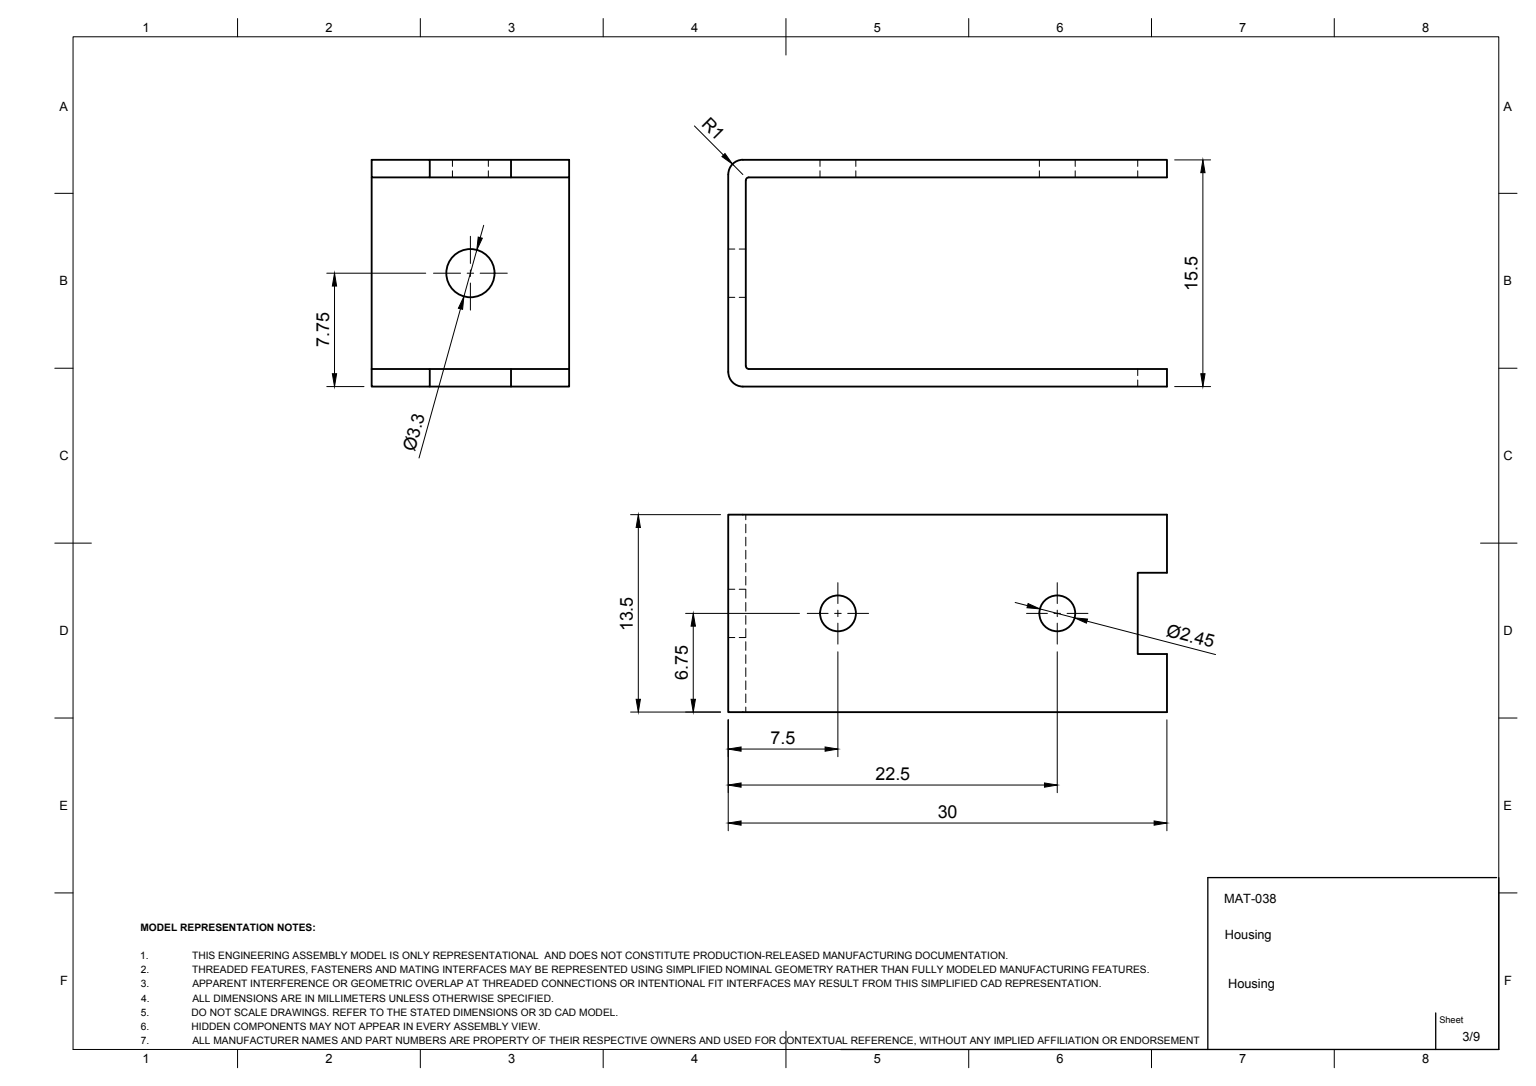
ISO-10303-21;
HEADER;
/* Generated by software containing ST-Developer
 * from STEP Tools, Inc. (www.steptools.com) 
 */

FILE_DESCRIPTION(
/* description */ ('STEP AP214'),
/* implementation_level */ '2;1');

FILE_NAME(
/* name */ 'Housing.step',
/* time_stamp */ '2026-11-14T21:32:33-08:00',
/* author */ (''),
/* organization */ (''),
/* preprocessor_version */ 'ST-DEVELOPER v20.2',
/* originating_system */ 'Autodesk Translation Framework v15.17.0.0',
/* authorisation */ '');

FILE_SCHEMA (('AUTOMOTIVE_DESIGN { 1 0 10303 214 3 1 1 }'));
ENDSEC;

DATA;
#10=MECHANICAL_DESIGN_GEOMETRIC_PRESENTATION_REPRESENTATION('',(#177),#10551);
#159=SHAPE_REPRESENTATION_RELATIONSHIP('SRR','None',#10586,#168);
#168=ADVANCED_BREP_SHAPE_REPRESENTATION('',(#187),#10542);
#177=STYLED_ITEM('',(#10640),#187);
#187=MANIFOLD_SOLID_BREP('Body1',#3426);
#197=FACE_BOUND('',#522,.T.);
#198=FACE_BOUND('',#523,.T.);
#199=FACE_BOUND('',#525,.T.);
#200=FACE_BOUND('',#531,.T.);
#201=FACE_BOUND('',#533,.T.);
#202=FACE_BOUND('',#534,.T.);
#224=PLANE('',#3547);
#225=PLANE('',#3548);
#226=PLANE('',#3549);
#227=PLANE('',#3550);
#228=PLANE('',#3551);
#229=PLANE('',#3552);
#230=PLANE('',#3553);
#231=PLANE('',#3554);
#232=PLANE('',#3559);
#233=PLANE('',#3564);
#234=PLANE('',#3565);
#235=PLANE('',#3566);
#236=PLANE('',#3571);
#237=PLANE('',#3572);
#238=PLANE('',#3573);
#239=PLANE('',#3574);
#240=PLANE('',#3575);
#241=PLANE('',#3576);
#294=FACE_OUTER_BOUND('',#514,.T.);
#295=FACE_OUTER_BOUND('',#515,.T.);
#296=FACE_OUTER_BOUND('',#516,.T.);
#297=FACE_OUTER_BOUND('',#517,.T.);
#298=FACE_OUTER_BOUND('',#518,.T.);
#299=FACE_OUTER_BOUND('',#519,.T.);
#300=FACE_OUTER_BOUND('',#520,.T.);
#301=FACE_OUTER_BOUND('',#521,.T.);
#302=FACE_OUTER_BOUND('',#524,.T.);
#303=FACE_OUTER_BOUND('',#526,.T.);
#304=FACE_OUTER_BOUND('',#527,.T.);
#305=FACE_OUTER_BOUND('',#528,.T.);
#306=FACE_OUTER_BOUND('',#529,.T.);
#307=FACE_OUTER_BOUND('',#530,.T.);
#308=FACE_OUTER_BOUND('',#532,.T.);
#309=FACE_OUTER_BOUND('',#535,.T.);
#310=FACE_OUTER_BOUND('',#536,.T.);
#311=FACE_OUTER_BOUND('',#537,.T.);
#312=FACE_OUTER_BOUND('',#538,.T.);
#313=FACE_OUTER_BOUND('',#539,.T.);
#314=FACE_OUTER_BOUND('',#540,.T.);
#315=FACE_OUTER_BOUND('',#541,.T.);
#316=FACE_OUTER_BOUND('',#542,.T.);
#317=FACE_OUTER_BOUND('',#543,.T.);
#318=FACE_OUTER_BOUND('',#544,.T.);
#514=EDGE_LOOP('',(#2188,#2189,#2190,#2191));
#515=EDGE_LOOP('',(#2192,#2193,#2194,#2195));
#516=EDGE_LOOP('',(#2196,#2197,#2198,#2199));
#517=EDGE_LOOP('',(#2200,#2201,#2202,#2203));
#518=EDGE_LOOP('',(#2204,#2205,#2206,#2207));
#519=EDGE_LOOP('',(#2208,#2209,#2210,#2211));
#520=EDGE_LOOP('',(#2212,#2213,#2214,#2215));
#521=EDGE_LOOP('',(#2216,#2217,#2218,#2219,#2220,#2221,#2222,#2223));
#522=EDGE_LOOP('',(#2224));
#523=EDGE_LOOP('',(#2225));
#524=EDGE_LOOP('',(#2226,#2227,#2228,#2229));
#525=EDGE_LOOP('',(#2230));
#526=EDGE_LOOP('',(#2231,#2232,#2233,#2234,#2235,#2236,#2237,#2238));
#527=EDGE_LOOP('',(#2239,#2240,#2241,#2242,#2243,#2244,#2245,#2246,#2247,
#2248,#2249,#2250));
#528=EDGE_LOOP('',(#2251,#2252,#2253,#2254,#2255,#2256,#2257,#2258,#2259,
#2260,#2261,#2262));
#529=EDGE_LOOP('',(#2263,#2264,#2265,#2266,#2267,#2268,#2269,#2270));
#530=EDGE_LOOP('',(#2271,#2272,#2273,#2274));
#531=EDGE_LOOP('',(#2275));
#532=EDGE_LOOP('',(#2276,#2277,#2278,#2279,#2280,#2281,#2282,#2283));
#533=EDGE_LOOP('',(#2284));
#534=EDGE_LOOP('',(#2285));
#535=EDGE_LOOP('',(#2286,#2287,#2288,#2289));
#536=EDGE_LOOP('',(#2290,#2291,#2292,#2293));
#537=EDGE_LOOP('',(#2294,#2295,#2296,#2297));
#538=EDGE_LOOP('',(#2298,#2299,#2300,#2301));
#539=EDGE_LOOP('',(#2302,#2303,#2304,#2305));
#540=EDGE_LOOP('',(#2306,#2307,#2308,#2309));
#541=EDGE_LOOP('',(#2310,#2311,#2312,#2313));
#542=EDGE_LOOP('',(#2314,#2315,#2316,#2317));
#543=EDGE_LOOP('',(#2318,#2319,#2320,#2321));
#544=EDGE_LOOP('',(#2322,#2323,#2324,#2325));
#761=LINE('',#5239,#958);
#762=LINE('',#5245,#959);
#763=LINE('',#5251,#960);
#764=LINE('',#5256,#961);
#765=LINE('',#5258,#962);
#766=LINE('',#5260,#963);
#767=LINE('',#5261,#964);
#768=LINE('',#5265,#965);
#769=LINE('',#5267,#966);
#770=LINE('',#5269,#967);
#771=LINE('',#5270,#968);
#772=LINE('',#5274,#969);
#773=LINE('',#5276,#970);
#774=LINE('',#5278,#971);
#775=LINE('',#5279,#972);
#776=LINE('',#5283,#973);
#777=LINE('',#5285,#974);
#778=LINE('',#5287,#975);
#779=LINE('',#5288,#976);
#780=LINE('',#5291,#977);
#781=LINE('',#5293,#978);
#782=LINE('',#5294,#979);
#783=LINE('',#5296,#980);
#784=LINE('',#5298,#981);
#785=LINE('',#5299,#982);
#786=LINE('',#5303,#983);
#787=LINE('',#5305,#984);
#788=LINE('',#5307,#985);
#789=LINE('',#5308,#986);
#790=LINE('',#5312,#987);
#791=LINE('',#5313,#988);
#792=LINE('',#5315,#989);
#793=LINE('',#5317,#990);
#794=LINE('',#5318,#991);
#795=LINE('',#5319,#992);
#796=LINE('',#5324,#993);
#797=LINE('',#5328,#994);
#798=LINE('',#5331,#995);
#799=LINE('',#5335,#996);
#800=LINE('',#5339,#997);
#801=LINE('',#5342,#998);
#802=LINE('',#5346,#999);
#803=LINE('',#5348,#1000);
#804=LINE('',#5349,#1001);
#805=LINE('',#5350,#1002);
#806=LINE('',#5352,#1003);
#807=LINE('',#5353,#1004);
#808=LINE('',#5357,#1005);
#809=LINE('',#5358,#1006);
#810=LINE('',#5359,#1007);
#811=LINE('',#5360,#1008);
#812=LINE('',#5366,#1009);
#813=LINE('',#5368,#1010);
#814=LINE('',#5371,#1011);
#815=LINE('',#5373,#1012);
#958=VECTOR('',#4044,1.225);
#959=VECTOR('',#4051,1.225);
#960=VECTOR('',#4058,1.65);
#961=VECTOR('',#4063,1000.);
#962=VECTOR('',#4064,1000.);
#963=VECTOR('',#4065,1000.);
#964=VECTOR('',#4066,1000.);
#965=VECTOR('',#4069,1000.);
#966=VECTOR('',#4070,1000.);
#967=VECTOR('',#4071,1000.);
#968=VECTOR('',#4072,1000.);
#969=VECTOR('',#4075,1000.);
#970=VECTOR('',#4076,1000.);
#971=VECTOR('',#4077,1000.);
#972=VECTOR('',#4078,1000.);
#973=VECTOR('',#4081,1000.);
#974=VECTOR('',#4082,1000.);
#975=VECTOR('',#4083,1000.);
#976=VECTOR('',#4084,1000.);
#977=VECTOR('',#4087,1000.);
#978=VECTOR('',#4088,1000.);
#979=VECTOR('',#4089,1000.);
#980=VECTOR('',#4090,1000.);
#981=VECTOR('',#4091,1000.);
#982=VECTOR('',#4092,1000.);
#983=VECTOR('',#4095,1000.);
#984=VECTOR('',#4096,1000.);
#985=VECTOR('',#4097,1000.);
#986=VECTOR('',#4098,1000.);
#987=VECTOR('',#4101,1000.);
#988=VECTOR('',#4102,1000.);
#989=VECTOR('',#4103,1000.);
#990=VECTOR('',#4104,1000.);
#991=VECTOR('',#4105,1000.);
#992=VECTOR('',#4106,1000.);
#993=VECTOR('',#4113,1000.);
#994=VECTOR('',#4116,1000.);
#995=VECTOR('',#4119,1000.);
#996=VECTOR('',#4124,1000.);
#997=VECTOR('',#4127,1000.);
#998=VECTOR('',#4130,1000.);
#999=VECTOR('',#4135,1000.);
#1000=VECTOR('',#4136,1000.);
#1001=VECTOR('',#4137,1000.);
#1002=VECTOR('',#4138,1000.);
#1003=VECTOR('',#4141,1000.);
#1004=VECTOR('',#4142,1000.);
#1005=VECTOR('',#4145,1000.);
#1006=VECTOR('',#4146,1000.);
#1007=VECTOR('',#4147,1000.);
#1008=VECTOR('',#4148,1000.);
#1009=VECTOR('',#4159,1000.);
#1010=VECTOR('',#4162,1000.);
#1011=VECTOR('',#4167,1000.);
#1012=VECTOR('',#4170,1000.);
#1155=CIRCLE('',#3539,1.225);
#1156=CIRCLE('',#3540,1.225);
#1157=CIRCLE('',#3542,1.225);
#1158=CIRCLE('',#3543,1.225);
#1159=CIRCLE('',#3545,1.65);
#1160=CIRCLE('',#3546,1.65);
#1161=CIRCLE('',#3555,1.);
#1162=CIRCLE('',#3556,1.);
#1163=CIRCLE('',#3557,0.2);
#1164=CIRCLE('',#3558,0.2);
#1165=CIRCLE('',#3560,1.);
#1166=CIRCLE('',#3561,0.2);
#1167=CIRCLE('',#3562,0.2);
#1168=CIRCLE('',#3563,1.);
#1421=VERTEX_POINT('',#5236);
#1422=VERTEX_POINT('',#5238);
#1423=VERTEX_POINT('',#5242);
#1424=VERTEX_POINT('',#5244);
#1425=VERTEX_POINT('',#5248);
#1426=VERTEX_POINT('',#5250);
#1427=VERTEX_POINT('',#5254);
#1428=VERTEX_POINT('',#5255);
#1429=VERTEX_POINT('',#5257);
#1430=VERTEX_POINT('',#5259);
#1431=VERTEX_POINT('',#5263);
#1432=VERTEX_POINT('',#5264);
#1433=VERTEX_POINT('',#5266);
#1434=VERTEX_POINT('',#5268);
#1435=VERTEX_POINT('',#5272);
#1436=VERTEX_POINT('',#5273);
#1437=VERTEX_POINT('',#5275);
#1438=VERTEX_POINT('',#5277);
#1439=VERTEX_POINT('',#5281);
#1440=VERTEX_POINT('',#5282);
#1441=VERTEX_POINT('',#5284);
#1442=VERTEX_POINT('',#5286);
#1443=VERTEX_POINT('',#5290);
#1444=VERTEX_POINT('',#5292);
#1445=VERTEX_POINT('',#5295);
#1446=VERTEX_POINT('',#5297);
#1447=VERTEX_POINT('',#5301);
#1448=VERTEX_POINT('',#5302);
#1449=VERTEX_POINT('',#5304);
#1450=VERTEX_POINT('',#5306);
#1451=VERTEX_POINT('',#5310);
#1452=VERTEX_POINT('',#5311);
#1453=VERTEX_POINT('',#5314);
#1454=VERTEX_POINT('',#5316);
#1455=VERTEX_POINT('',#5323);
#1456=VERTEX_POINT('',#5325);
#1457=VERTEX_POINT('',#5327);
#1458=VERTEX_POINT('',#5329);
#1459=VERTEX_POINT('',#5334);
#1460=VERTEX_POINT('',#5336);
#1461=VERTEX_POINT('',#5338);
#1462=VERTEX_POINT('',#5340);
#1463=VERTEX_POINT('',#5345);
#1464=VERTEX_POINT('',#5347);
#1465=VERTEX_POINT('',#5355);
#1466=VERTEX_POINT('',#5356);
#1707=EDGE_CURVE('',#1421,#1421,#1155,.T.);
#1708=EDGE_CURVE('',#1421,#1422,#761,.T.);
#1709=EDGE_CURVE('',#1422,#1422,#1156,.T.);
#1710=EDGE_CURVE('',#1423,#1423,#1157,.T.);
#1711=EDGE_CURVE('',#1423,#1424,#762,.T.);
#1712=EDGE_CURVE('',#1424,#1424,#1158,.T.);
#1713=EDGE_CURVE('',#1425,#1425,#1159,.T.);
#1714=EDGE_CURVE('',#1425,#1426,#763,.T.);
#1715=EDGE_CURVE('',#1426,#1426,#1160,.T.);
#1716=EDGE_CURVE('',#1427,#1428,#764,.T.);
#1717=EDGE_CURVE('',#1428,#1429,#765,.T.);
#1718=EDGE_CURVE('',#1429,#1430,#766,.T.);
#1719=EDGE_CURVE('',#1427,#1430,#767,.T.);
#1720=EDGE_CURVE('',#1431,#1432,#768,.T.);
#1721=EDGE_CURVE('',#1431,#1433,#769,.T.);
#1722=EDGE_CURVE('',#1434,#1433,#770,.T.);
#1723=EDGE_CURVE('',#1432,#1434,#771,.T.);
#1724=EDGE_CURVE('',#1435,#1436,#772,.T.);
#1725=EDGE_CURVE('',#1437,#1436,#773,.T.);
#1726=EDGE_CURVE('',#1437,#1438,#774,.T.);
#1727=EDGE_CURVE('',#1438,#1435,#775,.T.);
#1728=EDGE_CURVE('',#1439,#1440,#776,.T.);
#1729=EDGE_CURVE('',#1441,#1439,#777,.T.);
#1730=EDGE_CURVE('',#1442,#1441,#778,.T.);
#1731=EDGE_CURVE('',#1442,#1440,#779,.T.);
#1732=EDGE_CURVE('',#1443,#1433,#780,.T.);
#1733=EDGE_CURVE('',#1444,#1443,#781,.T.);
#1734=EDGE_CURVE('',#1439,#1444,#782,.T.);
#1735=EDGE_CURVE('',#1440,#1445,#783,.T.);
#1736=EDGE_CURVE('',#1445,#1446,#784,.T.);
#1737=EDGE_CURVE('',#1434,#1446,#785,.T.);
#1738=EDGE_CURVE('',#1447,#1448,#786,.T.);
#1739=EDGE_CURVE('',#1447,#1449,#787,.T.);
#1740=EDGE_CURVE('',#1449,#1450,#788,.T.);
#1741=EDGE_CURVE('',#1450,#1448,#789,.T.);
#1742=EDGE_CURVE('',#1451,#1452,#790,.T.);
#1743=EDGE_CURVE('',#1452,#1428,#791,.T.);
#1744=EDGE_CURVE('',#1453,#1427,#792,.T.);
#1745=EDGE_CURVE('',#1453,#1454,#793,.T.);
#1746=EDGE_CURVE('',#1454,#1438,#794,.T.);
#1747=EDGE_CURVE('',#1437,#1451,#795,.T.);
#1748=EDGE_CURVE('',#1446,#1447,#1161,.T.);
#1749=EDGE_CURVE('',#1448,#1453,#1162,.T.);
#1750=EDGE_CURVE('',#1455,#1430,#796,.T.);
#1751=EDGE_CURVE('',#1455,#1456,#1163,.T.);
#1752=EDGE_CURVE('',#1457,#1456,#797,.T.);
#1753=EDGE_CURVE('',#1457,#1458,#1164,.T.);
#1754=EDGE_CURVE('',#1432,#1458,#798,.T.);
#1755=EDGE_CURVE('',#1449,#1445,#1165,.T.);
#1756=EDGE_CURVE('',#1442,#1459,#799,.T.);
#1757=EDGE_CURVE('',#1459,#1460,#1166,.T.);
#1758=EDGE_CURVE('',#1460,#1461,#800,.T.);
#1759=EDGE_CURVE('',#1461,#1462,#1167,.T.);
#1760=EDGE_CURVE('',#1462,#1435,#801,.T.);
#1761=EDGE_CURVE('',#1454,#1450,#1168,.T.);
#1762=EDGE_CURVE('',#1429,#1463,#802,.T.);
#1763=EDGE_CURVE('',#1463,#1464,#803,.T.);
#1764=EDGE_CURVE('',#1464,#1436,#804,.T.);
#1765=EDGE_CURVE('',#1462,#1455,#805,.T.);
#1766=EDGE_CURVE('',#1460,#1457,#806,.T.);
#1767=EDGE_CURVE('',#1456,#1461,#807,.T.);
#1768=EDGE_CURVE('',#1465,#1466,#808,.T.);
#1769=EDGE_CURVE('',#1466,#1431,#809,.T.);
#1770=EDGE_CURVE('',#1458,#1459,#810,.T.);
#1771=EDGE_CURVE('',#1441,#1465,#811,.T.);
#1772=EDGE_CURVE('',#1465,#1444,#812,.T.);
#1773=EDGE_CURVE('',#1466,#1443,#813,.T.);
#1774=EDGE_CURVE('',#1452,#1463,#814,.T.);
#1775=EDGE_CURVE('',#1451,#1464,#815,.T.);
#2188=ORIENTED_EDGE('',*,*,#1707,.T.);
#2189=ORIENTED_EDGE('',*,*,#1708,.T.);
#2190=ORIENTED_EDGE('',*,*,#1709,.T.);
#2191=ORIENTED_EDGE('',*,*,#1708,.F.);
#2192=ORIENTED_EDGE('',*,*,#1710,.T.);
#2193=ORIENTED_EDGE('',*,*,#1711,.T.);
#2194=ORIENTED_EDGE('',*,*,#1712,.T.);
#2195=ORIENTED_EDGE('',*,*,#1711,.F.);
#2196=ORIENTED_EDGE('',*,*,#1713,.T.);
#2197=ORIENTED_EDGE('',*,*,#1714,.T.);
#2198=ORIENTED_EDGE('',*,*,#1715,.T.);
#2199=ORIENTED_EDGE('',*,*,#1714,.F.);
#2200=ORIENTED_EDGE('',*,*,#1716,.T.);
#2201=ORIENTED_EDGE('',*,*,#1717,.T.);
#2202=ORIENTED_EDGE('',*,*,#1718,.T.);
#2203=ORIENTED_EDGE('',*,*,#1719,.F.);
#2204=ORIENTED_EDGE('',*,*,#1720,.F.);
#2205=ORIENTED_EDGE('',*,*,#1721,.T.);
#2206=ORIENTED_EDGE('',*,*,#1722,.F.);
#2207=ORIENTED_EDGE('',*,*,#1723,.F.);
#2208=ORIENTED_EDGE('',*,*,#1724,.T.);
#2209=ORIENTED_EDGE('',*,*,#1725,.F.);
#2210=ORIENTED_EDGE('',*,*,#1726,.T.);
#2211=ORIENTED_EDGE('',*,*,#1727,.T.);
#2212=ORIENTED_EDGE('',*,*,#1728,.F.);
#2213=ORIENTED_EDGE('',*,*,#1729,.F.);
#2214=ORIENTED_EDGE('',*,*,#1730,.F.);
#2215=ORIENTED_EDGE('',*,*,#1731,.T.);
#2216=ORIENTED_EDGE('',*,*,#1722,.T.);
#2217=ORIENTED_EDGE('',*,*,#1732,.F.);
#2218=ORIENTED_EDGE('',*,*,#1733,.F.);
#2219=ORIENTED_EDGE('',*,*,#1734,.F.);
#2220=ORIENTED_EDGE('',*,*,#1728,.T.);
#2221=ORIENTED_EDGE('',*,*,#1735,.T.);
#2222=ORIENTED_EDGE('',*,*,#1736,.T.);
#2223=ORIENTED_EDGE('',*,*,#1737,.F.);
#2224=ORIENTED_EDGE('',*,*,#1709,.F.);
#2225=ORIENTED_EDGE('',*,*,#1712,.F.);
#2226=ORIENTED_EDGE('',*,*,#1738,.F.);
#2227=ORIENTED_EDGE('',*,*,#1739,.T.);
#2228=ORIENTED_EDGE('',*,*,#1740,.T.);
#2229=ORIENTED_EDGE('',*,*,#1741,.T.);
#2230=ORIENTED_EDGE('',*,*,#1715,.F.);
#2231=ORIENTED_EDGE('',*,*,#1742,.T.);
#2232=ORIENTED_EDGE('',*,*,#1743,.T.);
#2233=ORIENTED_EDGE('',*,*,#1716,.F.);
#2234=ORIENTED_EDGE('',*,*,#1744,.F.);
#2235=ORIENTED_EDGE('',*,*,#1745,.T.);
#2236=ORIENTED_EDGE('',*,*,#1746,.T.);
#2237=ORIENTED_EDGE('',*,*,#1726,.F.);
#2238=ORIENTED_EDGE('',*,*,#1747,.T.);
#2239=ORIENTED_EDGE('',*,*,#1737,.T.);
#2240=ORIENTED_EDGE('',*,*,#1748,.T.);
#2241=ORIENTED_EDGE('',*,*,#1738,.T.);
#2242=ORIENTED_EDGE('',*,*,#1749,.T.);
#2243=ORIENTED_EDGE('',*,*,#1744,.T.);
#2244=ORIENTED_EDGE('',*,*,#1719,.T.);
#2245=ORIENTED_EDGE('',*,*,#1750,.F.);
#2246=ORIENTED_EDGE('',*,*,#1751,.T.);
#2247=ORIENTED_EDGE('',*,*,#1752,.F.);
#2248=ORIENTED_EDGE('',*,*,#1753,.T.);
#2249=ORIENTED_EDGE('',*,*,#1754,.F.);
#2250=ORIENTED_EDGE('',*,*,#1723,.T.);
#2251=ORIENTED_EDGE('',*,*,#1740,.F.);
#2252=ORIENTED_EDGE('',*,*,#1755,.T.);
#2253=ORIENTED_EDGE('',*,*,#1735,.F.);
#2254=ORIENTED_EDGE('',*,*,#1731,.F.);
#2255=ORIENTED_EDGE('',*,*,#1756,.T.);
#2256=ORIENTED_EDGE('',*,*,#1757,.T.);
#2257=ORIENTED_EDGE('',*,*,#1758,.T.);
#2258=ORIENTED_EDGE('',*,*,#1759,.T.);
#2259=ORIENTED_EDGE('',*,*,#1760,.T.);
#2260=ORIENTED_EDGE('',*,*,#1727,.F.);
#2261=ORIENTED_EDGE('',*,*,#1746,.F.);
#2262=ORIENTED_EDGE('',*,*,#1761,.T.);
#2263=ORIENTED_EDGE('',*,*,#1718,.F.);
#2264=ORIENTED_EDGE('',*,*,#1762,.T.);
#2265=ORIENTED_EDGE('',*,*,#1763,.T.);
#2266=ORIENTED_EDGE('',*,*,#1764,.T.);
#2267=ORIENTED_EDGE('',*,*,#1724,.F.);
#2268=ORIENTED_EDGE('',*,*,#1760,.F.);
#2269=ORIENTED_EDGE('',*,*,#1765,.T.);
#2270=ORIENTED_EDGE('',*,*,#1750,.T.);
#2271=ORIENTED_EDGE('',*,*,#1758,.F.);
#2272=ORIENTED_EDGE('',*,*,#1766,.T.);
#2273=ORIENTED_EDGE('',*,*,#1752,.T.);
#2274=ORIENTED_EDGE('',*,*,#1767,.T.);
#2275=ORIENTED_EDGE('',*,*,#1713,.F.);
#2276=ORIENTED_EDGE('',*,*,#1768,.T.);
#2277=ORIENTED_EDGE('',*,*,#1769,.T.);
#2278=ORIENTED_EDGE('',*,*,#1720,.T.);
#2279=ORIENTED_EDGE('',*,*,#1754,.T.);
#2280=ORIENTED_EDGE('',*,*,#1770,.T.);
#2281=ORIENTED_EDGE('',*,*,#1756,.F.);
#2282=ORIENTED_EDGE('',*,*,#1730,.T.);
#2283=ORIENTED_EDGE('',*,*,#1771,.T.);
#2284=ORIENTED_EDGE('',*,*,#1707,.F.);
#2285=ORIENTED_EDGE('',*,*,#1710,.F.);
#2286=ORIENTED_EDGE('',*,*,#1748,.F.);
#2287=ORIENTED_EDGE('',*,*,#1736,.F.);
#2288=ORIENTED_EDGE('',*,*,#1755,.F.);
#2289=ORIENTED_EDGE('',*,*,#1739,.F.);
#2290=ORIENTED_EDGE('',*,*,#1749,.F.);
#2291=ORIENTED_EDGE('',*,*,#1741,.F.);
#2292=ORIENTED_EDGE('',*,*,#1761,.F.);
#2293=ORIENTED_EDGE('',*,*,#1745,.F.);
#2294=ORIENTED_EDGE('',*,*,#1757,.F.);
#2295=ORIENTED_EDGE('',*,*,#1770,.F.);
#2296=ORIENTED_EDGE('',*,*,#1753,.F.);
#2297=ORIENTED_EDGE('',*,*,#1766,.F.);
#2298=ORIENTED_EDGE('',*,*,#1759,.F.);
#2299=ORIENTED_EDGE('',*,*,#1767,.F.);
#2300=ORIENTED_EDGE('',*,*,#1751,.F.);
#2301=ORIENTED_EDGE('',*,*,#1765,.F.);
#2302=ORIENTED_EDGE('',*,*,#1729,.T.);
#2303=ORIENTED_EDGE('',*,*,#1734,.T.);
#2304=ORIENTED_EDGE('',*,*,#1772,.F.);
#2305=ORIENTED_EDGE('',*,*,#1771,.F.);
#2306=ORIENTED_EDGE('',*,*,#1772,.T.);
#2307=ORIENTED_EDGE('',*,*,#1733,.T.);
#2308=ORIENTED_EDGE('',*,*,#1773,.F.);
#2309=ORIENTED_EDGE('',*,*,#1768,.F.);
#2310=ORIENTED_EDGE('',*,*,#1773,.T.);
#2311=ORIENTED_EDGE('',*,*,#1732,.T.);
#2312=ORIENTED_EDGE('',*,*,#1721,.F.);
#2313=ORIENTED_EDGE('',*,*,#1769,.F.);
#2314=ORIENTED_EDGE('',*,*,#1717,.F.);
#2315=ORIENTED_EDGE('',*,*,#1743,.F.);
#2316=ORIENTED_EDGE('',*,*,#1774,.T.);
#2317=ORIENTED_EDGE('',*,*,#1762,.F.);
#2318=ORIENTED_EDGE('',*,*,#1774,.F.);
#2319=ORIENTED_EDGE('',*,*,#1742,.F.);
#2320=ORIENTED_EDGE('',*,*,#1775,.T.);
#2321=ORIENTED_EDGE('',*,*,#1763,.F.);
#2322=ORIENTED_EDGE('',*,*,#1775,.F.);
#2323=ORIENTED_EDGE('',*,*,#1747,.F.);
#2324=ORIENTED_EDGE('',*,*,#1725,.T.);
#2325=ORIENTED_EDGE('',*,*,#1764,.F.);
#3150=CYLINDRICAL_SURFACE('',#3538,1.225);
#3151=CYLINDRICAL_SURFACE('',#3541,1.225);
#3152=CYLINDRICAL_SURFACE('',#3544,1.65);
#3153=CYLINDRICAL_SURFACE('',#3567,1.);
#3154=CYLINDRICAL_SURFACE('',#3568,1.);
#3155=CYLINDRICAL_SURFACE('',#3569,0.2);
#3156=CYLINDRICAL_SURFACE('',#3570,0.2);
#3206=ADVANCED_FACE('',(#294),#3150,.F.);
#3207=ADVANCED_FACE('',(#295),#3151,.F.);
#3208=ADVANCED_FACE('',(#296),#3152,.F.);
#3209=ADVANCED_FACE('',(#297),#224,.F.);
#3210=ADVANCED_FACE('',(#298),#225,.F.);
#3211=ADVANCED_FACE('',(#299),#226,.F.);
#3212=ADVANCED_FACE('',(#300),#227,.F.);
#3213=ADVANCED_FACE('',(#301,#197,#198),#228,.F.);
#3214=ADVANCED_FACE('',(#302,#199),#229,.F.);
#3215=ADVANCED_FACE('',(#303),#230,.F.);
#3216=ADVANCED_FACE('',(#304),#231,.T.);
#3217=ADVANCED_FACE('',(#305),#232,.F.);
#3218=ADVANCED_FACE('',(#306),#233,.F.);
#3219=ADVANCED_FACE('',(#307,#200),#234,.F.);
#3220=ADVANCED_FACE('',(#308,#201,#202),#235,.F.);
#3221=ADVANCED_FACE('',(#309),#3153,.T.);
#3222=ADVANCED_FACE('',(#310),#3154,.T.);
#3223=ADVANCED_FACE('',(#311),#3155,.F.);
#3224=ADVANCED_FACE('',(#312),#3156,.F.);
#3225=ADVANCED_FACE('',(#313),#236,.F.);
#3226=ADVANCED_FACE('',(#314),#237,.F.);
#3227=ADVANCED_FACE('',(#315),#238,.F.);
#3228=ADVANCED_FACE('',(#316),#239,.F.);
#3229=ADVANCED_FACE('',(#317),#240,.F.);
#3230=ADVANCED_FACE('',(#318),#241,.F.);
#3426=CLOSED_SHELL('',(#3206,#3207,#3208,#3209,#3210,#3211,#3212,#3213,
#3214,#3215,#3216,#3217,#3218,#3219,#3220,#3221,#3222,#3223,#3224,#3225,
#3226,#3227,#3228,#3229,#3230));
#3537=AXIS2_PLACEMENT_3D('',#5234,#4038,#4039);
#3538=AXIS2_PLACEMENT_3D('',#5235,#4040,#4041);
#3539=AXIS2_PLACEMENT_3D('',#5237,#4042,#4043);
#3540=AXIS2_PLACEMENT_3D('',#5240,#4045,#4046);
#3541=AXIS2_PLACEMENT_3D('',#5241,#4047,#4048);
#3542=AXIS2_PLACEMENT_3D('',#5243,#4049,#4050);
#3543=AXIS2_PLACEMENT_3D('',#5246,#4052,#4053);
#3544=AXIS2_PLACEMENT_3D('',#5247,#4054,#4055);
#3545=AXIS2_PLACEMENT_3D('',#5249,#4056,#4057);
#3546=AXIS2_PLACEMENT_3D('',#5252,#4059,#4060);
#3547=AXIS2_PLACEMENT_3D('',#5253,#4061,#4062);
#3548=AXIS2_PLACEMENT_3D('',#5262,#4067,#4068);
#3549=AXIS2_PLACEMENT_3D('',#5271,#4073,#4074);
#3550=AXIS2_PLACEMENT_3D('',#5280,#4079,#4080);
#3551=AXIS2_PLACEMENT_3D('',#5289,#4085,#4086);
#3552=AXIS2_PLACEMENT_3D('',#5300,#4093,#4094);
#3553=AXIS2_PLACEMENT_3D('',#5309,#4099,#4100);
#3554=AXIS2_PLACEMENT_3D('',#5320,#4107,#4108);
#3555=AXIS2_PLACEMENT_3D('',#5321,#4109,#4110);
#3556=AXIS2_PLACEMENT_3D('',#5322,#4111,#4112);
#3557=AXIS2_PLACEMENT_3D('',#5326,#4114,#4115);
#3558=AXIS2_PLACEMENT_3D('',#5330,#4117,#4118);
#3559=AXIS2_PLACEMENT_3D('',#5332,#4120,#4121);
#3560=AXIS2_PLACEMENT_3D('',#5333,#4122,#4123);
#3561=AXIS2_PLACEMENT_3D('',#5337,#4125,#4126);
#3562=AXIS2_PLACEMENT_3D('',#5341,#4128,#4129);
#3563=AXIS2_PLACEMENT_3D('',#5343,#4131,#4132);
#3564=AXIS2_PLACEMENT_3D('',#5344,#4133,#4134);
#3565=AXIS2_PLACEMENT_3D('',#5351,#4139,#4140);
#3566=AXIS2_PLACEMENT_3D('',#5354,#4143,#4144);
#3567=AXIS2_PLACEMENT_3D('',#5361,#4149,#4150);
#3568=AXIS2_PLACEMENT_3D('',#5362,#4151,#4152);
#3569=AXIS2_PLACEMENT_3D('',#5363,#4153,#4154);
#3570=AXIS2_PLACEMENT_3D('',#5364,#4155,#4156);
#3571=AXIS2_PLACEMENT_3D('',#5365,#4157,#4158);
#3572=AXIS2_PLACEMENT_3D('',#5367,#4160,#4161);
#3573=AXIS2_PLACEMENT_3D('',#5369,#4163,#4164);
#3574=AXIS2_PLACEMENT_3D('',#5370,#4165,#4166);
#3575=AXIS2_PLACEMENT_3D('',#5372,#4168,#4169);
#3576=AXIS2_PLACEMENT_3D('',#5374,#4171,#4172);
#4038=DIRECTION('axis',(0.,0.,1.));
#4039=DIRECTION('refdir',(1.,0.,0.));
#4040=DIRECTION('center_axis',(0.,0.,1.));
#4041=DIRECTION('ref_axis',(1.,0.,0.));
#4042=DIRECTION('center_axis',(-3.61400724161835E-16,0.,-1.));
#4043=DIRECTION('ref_axis',(1.,0.,-3.61400724161835E-16));
#4044=DIRECTION('',(0.,0.,1.));
#4045=DIRECTION('center_axis',(0.,0.,1.));
#4046=DIRECTION('ref_axis',(1.,0.,0.));
#4047=DIRECTION('center_axis',(0.,0.,1.));
#4048=DIRECTION('ref_axis',(1.,0.,0.));
#4049=DIRECTION('center_axis',(-3.61400724161835E-16,0.,-1.));
#4050=DIRECTION('ref_axis',(1.,0.,-3.61400724161835E-16));
#4051=DIRECTION('',(0.,0.,1.));
#4052=DIRECTION('center_axis',(0.,0.,1.));
#4053=DIRECTION('ref_axis',(1.,0.,0.));
#4054=DIRECTION('center_axis',(1.,0.,-2.23835287222814E-16));
#4055=DIRECTION('ref_axis',(-2.23835287222814E-16,0.,-1.));
#4056=DIRECTION('center_axis',(-1.,0.,1.32421639387543E-16));
#4057=DIRECTION('ref_axis',(-1.32421639387543E-16,0.,-1.));
#4058=DIRECTION('',(1.,0.,-2.23835287222814E-16));
#4059=DIRECTION('center_axis',(1.,0.,-2.23835287222814E-16));
#4060=DIRECTION('ref_axis',(-2.23835287222814E-16,0.,-1.));
#4061=DIRECTION('center_axis',(1.,0.,-3.35752930834221E-16));
#4062=DIRECTION('ref_axis',(-3.35752930834221E-16,0.,-1.));
#4063=DIRECTION('',(0.,-1.,0.));
#4064=DIRECTION('',(0.,0.,1.));
#4065=DIRECTION('',(0.,1.,0.));
#4066=DIRECTION('',(3.35752930834221E-16,0.,1.));
#4067=DIRECTION('center_axis',(1.,0.,-3.35752930834221E-16));
#4068=DIRECTION('ref_axis',(-3.35752930834221E-16,0.,-1.));
#4069=DIRECTION('',(0.,1.,0.));
#4070=DIRECTION('',(0.,0.,1.));
#4071=DIRECTION('',(0.,-1.,0.));
#4072=DIRECTION('',(3.35752930834221E-16,0.,1.));
#4073=DIRECTION('center_axis',(1.,0.,-3.35752930834221E-16));
#4074=DIRECTION('ref_axis',(-3.35752930834221E-16,0.,-1.));
#4075=DIRECTION('',(0.,1.,0.));
#4076=DIRECTION('',(0.,0.,1.));
#4077=DIRECTION('',(0.,-1.,0.));
#4078=DIRECTION('',(3.35752930834221E-16,0.,1.));
#4079=DIRECTION('center_axis',(1.,0.,-3.35752930834221E-16));
#4080=DIRECTION('ref_axis',(-3.35752930834221E-16,0.,-1.));
#4081=DIRECTION('',(0.,-1.,0.));
#4082=DIRECTION('',(0.,0.,1.));
#4083=DIRECTION('',(0.,1.,0.));
#4084=DIRECTION('',(3.35752930834221E-16,0.,1.));
#4085=DIRECTION('center_axis',(0.,0.,-1.));
#4086=DIRECTION('ref_axis',(-1.,0.,0.));
#4087=DIRECTION('',(-1.,-4.33680868994202E-16,0.));
#4088=DIRECTION('',(-3.1256278846429E-16,1.,0.));
#4089=DIRECTION('',(1.,0.,0.));
#4090=DIRECTION('',(1.,0.,0.));
#4091=DIRECTION('',(0.,1.,0.));
#4092=DIRECTION('',(1.,0.,0.));
#4093=DIRECTION('center_axis',(-1.,0.,2.23835287222814E-16));
#4094=DIRECTION('ref_axis',(2.23835287222814E-16,0.,1.));
#4095=DIRECTION('',(-2.23835287222814E-16,0.,-1.));
#4096=DIRECTION('',(0.,-1.,0.));
#4097=DIRECTION('',(-2.23835287222814E-16,0.,-1.));
#4098=DIRECTION('',(0.,1.,0.));
#4099=DIRECTION('center_axis',(0.,0.,1.));
#4100=DIRECTION('ref_axis',(1.,0.,0.));
#4101=DIRECTION('',(-3.1256278846429E-16,1.,0.));
#4102=DIRECTION('',(-1.,-4.33680868994202E-16,0.));
#4103=DIRECTION('',(-1.,0.,0.));
#4104=DIRECTION('',(0.,-1.,0.));
#4105=DIRECTION('',(-1.,0.,0.));
#4106=DIRECTION('',(1.,0.,0.));
#4107=DIRECTION('center_axis',(0.,1.,0.));
#4108=DIRECTION('ref_axis',(0.,0.,1.));
#4109=DIRECTION('center_axis',(0.,1.,0.));
#4110=DIRECTION('ref_axis',(0.,0.,1.));
#4111=DIRECTION('center_axis',(0.,1.,0.));
#4112=DIRECTION('ref_axis',(0.,0.,1.));
#4113=DIRECTION('',(-1.,0.,0.));
#4114=DIRECTION('center_axis',(0.,-1.,0.));
#4115=DIRECTION('ref_axis',(0.,0.,1.));
#4116=DIRECTION('',(-1.32421639387543E-16,0.,-1.));
#4117=DIRECTION('center_axis',(0.,-1.,0.));
#4118=DIRECTION('ref_axis',(2.60208521396522E-14,0.,1.));
#4119=DIRECTION('',(1.,0.,-3.61400724161835E-16));
#4120=DIRECTION('center_axis',(0.,1.,0.));
#4121=DIRECTION('ref_axis',(0.,0.,1.));
#4122=DIRECTION('center_axis',(0.,-1.,0.));
#4123=DIRECTION('ref_axis',(5.20417042793042E-15,0.,1.));
#4124=DIRECTION('',(1.,0.,-3.61400724161835E-16));
#4125=DIRECTION('center_axis',(0.,1.,0.));
#4126=DIRECTION('ref_axis',(0.,0.,1.));
#4127=DIRECTION('',(-1.32421639387543E-16,0.,-1.));
#4128=DIRECTION('center_axis',(0.,1.,0.));
#4129=DIRECTION('ref_axis',(0.,0.,1.));
#4130=DIRECTION('',(-1.,0.,0.));
#4131=DIRECTION('center_axis',(0.,-1.,0.));
#4132=DIRECTION('ref_axis',(0.,0.,1.));
#4133=DIRECTION('center_axis',(0.,0.,-1.));
#4134=DIRECTION('ref_axis',(-1.,0.,0.));
#4135=DIRECTION('',(1.,4.33680868994202E-16,0.));
#4136=DIRECTION('',(3.1256278846429E-16,-1.,0.));
#4137=DIRECTION('',(-1.,0.,0.));
#4138=DIRECTION('',(0.,1.,0.));
#4139=DIRECTION('center_axis',(1.,0.,-1.32421639387543E-16));
#4140=DIRECTION('ref_axis',(-1.32421639387543E-16,0.,-1.));
#4141=DIRECTION('',(0.,1.,0.));
#4142=DIRECTION('',(0.,-1.,0.));
#4143=DIRECTION('center_axis',(3.61400724161835E-16,0.,1.));
#4144=DIRECTION('ref_axis',(1.,0.,-3.61400724161835E-16));
#4145=DIRECTION('',(-3.1256278846429E-16,1.,1.12960418097037E-31));
#4146=DIRECTION('',(-1.,-4.33680868994202E-16,3.61400724161835E-16));
#4147=DIRECTION('',(0.,-1.,0.));
#4148=DIRECTION('',(1.,0.,-3.61400724161835E-16));
#4149=DIRECTION('center_axis',(0.,-1.,0.));
#4150=DIRECTION('ref_axis',(0.,0.,-1.));
#4151=DIRECTION('center_axis',(0.,-1.,0.));
#4152=DIRECTION('ref_axis',(0.,0.,-1.));
#4153=DIRECTION('center_axis',(0.,-1.,0.));
#4154=DIRECTION('ref_axis',(0.,0.,-1.));
#4155=DIRECTION('center_axis',(0.,-1.,0.));
#4156=DIRECTION('ref_axis',(0.,0.,-1.));
#4157=DIRECTION('center_axis',(0.,-1.,0.));
#4158=DIRECTION('ref_axis',(0.,0.,-1.));
#4159=DIRECTION('',(0.,0.,1.));
#4160=DIRECTION('center_axis',(1.,3.1256278846429E-16,0.));
#4161=DIRECTION('ref_axis',(-3.1256278846429E-16,1.,0.));
#4162=DIRECTION('',(0.,0.,1.));
#4163=DIRECTION('center_axis',(-4.33680868994202E-16,1.,0.));
#4164=DIRECTION('ref_axis',(-1.,-4.33680868994202E-16,0.));
#4165=DIRECTION('center_axis',(-4.33680868994202E-16,1.,0.));
#4166=DIRECTION('ref_axis',(-1.,-4.33680868994202E-16,0.));
#4167=DIRECTION('',(0.,0.,1.));
#4168=DIRECTION('center_axis',(1.,3.1256278846429E-16,0.));
#4169=DIRECTION('ref_axis',(-3.1256278846429E-16,1.,0.));
#4170=DIRECTION('',(0.,0.,1.));
#4171=DIRECTION('center_axis',(0.,-1.,0.));
#4172=DIRECTION('ref_axis',(0.,0.,-1.));
#5234=CARTESIAN_POINT('',(0.,0.,0.));
#5235=CARTESIAN_POINT('Origin',(7.50000000000001,0.,-7.751));
#5236=CARTESIAN_POINT('',(6.275,-1.50019232895551E-16,6.54999999999999));
#5237=CARTESIAN_POINT('Origin',(7.50000000000001,0.,6.54999999999999));
#5238=CARTESIAN_POINT('',(6.275,-1.50019232895551E-16,7.75));
#5239=CARTESIAN_POINT('',(6.275,-1.50019232895551E-16,-7.751));
#5240=CARTESIAN_POINT('Origin',(7.50000000000001,0.,7.75));
#5241=CARTESIAN_POINT('Origin',(-7.5,0.,-7.751));
#5242=CARTESIAN_POINT('',(-8.725,-1.50019232895551E-16,6.55));
#5243=CARTESIAN_POINT('Origin',(-7.5,0.,6.55));
#5244=CARTESIAN_POINT('',(-8.725,-1.50019232895551E-16,7.75));
#5245=CARTESIAN_POINT('',(-8.725,-1.50019232895551E-16,-7.751));
#5246=CARTESIAN_POINT('Origin',(-7.5,0.,7.75));
#5247=CARTESIAN_POINT('Origin',(-15.001,0.,3.35775314362943E-15));
#5248=CARTESIAN_POINT('',(13.8,-2.02066721859313E-16,1.65));
#5249=CARTESIAN_POINT('Origin',(13.8,0.,-3.08892696367483E-15));
#5250=CARTESIAN_POINT('',(15.,-2.02066721859313E-16,1.65));
#5251=CARTESIAN_POINT('',(-15.001,-2.02066721859313E-16,1.65));
#5252=CARTESIAN_POINT('Origin',(15.,0.,-3.35752930834221E-15));
#5253=CARTESIAN_POINT('Origin',(-15.,6.75,-7.75));
#5254=CARTESIAN_POINT('',(-15.,6.75,-7.75));
#5255=CARTESIAN_POINT('',(-15.,2.775,-7.75));
#5256=CARTESIAN_POINT('',(-15.,6.75,-7.75));
#5257=CARTESIAN_POINT('',(-15.,2.775,-6.55));
#5258=CARTESIAN_POINT('',(-15.,2.775,-7.75));
#5259=CARTESIAN_POINT('',(-15.,6.75,-6.55));
#5260=CARTESIAN_POINT('',(-15.,-6.75,-6.55));
#5261=CARTESIAN_POINT('',(-15.,6.75,-7.75));
#5262=CARTESIAN_POINT('Origin',(-15.,6.75,-7.75));
#5263=CARTESIAN_POINT('',(-15.,2.775,6.55));
#5264=CARTESIAN_POINT('',(-15.,6.75,6.55));
#5265=CARTESIAN_POINT('',(-15.,-6.75,6.55));
#5266=CARTESIAN_POINT('',(-15.,2.775,7.75));
#5267=CARTESIAN_POINT('',(-15.,2.775,-7.75));
#5268=CARTESIAN_POINT('',(-15.,6.75,7.75));
#5269=CARTESIAN_POINT('',(-15.,6.75,7.75));
#5270=CARTESIAN_POINT('',(-15.,6.75,-7.75));
#5271=CARTESIAN_POINT('Origin',(-15.,6.75,-7.75));
#5272=CARTESIAN_POINT('',(-15.,-6.75,-6.55));
#5273=CARTESIAN_POINT('',(-15.,-2.775,-6.55));
#5274=CARTESIAN_POINT('',(-15.,-6.75,-6.55));
#5275=CARTESIAN_POINT('',(-15.,-2.775,-7.75));
#5276=CARTESIAN_POINT('',(-15.,-2.775,-7.75));
#5277=CARTESIAN_POINT('',(-15.,-6.75,-7.75));
#5278=CARTESIAN_POINT('',(-15.,6.75,-7.75));
#5279=CARTESIAN_POINT('',(-15.,-6.75,-7.75));
#5280=CARTESIAN_POINT('Origin',(-15.,6.75,-7.75));
#5281=CARTESIAN_POINT('',(-15.,-2.775,7.75));
#5282=CARTESIAN_POINT('',(-15.,-6.75,7.75));
#5283=CARTESIAN_POINT('',(-15.,6.75,7.75));
#5284=CARTESIAN_POINT('',(-15.,-2.775,6.55));
#5285=CARTESIAN_POINT('',(-15.,-2.775,-7.75));
#5286=CARTESIAN_POINT('',(-15.,-6.75,6.55));
#5287=CARTESIAN_POINT('',(-15.,-6.75,6.55));
#5288=CARTESIAN_POINT('',(-15.,-6.75,-7.75));
#5289=CARTESIAN_POINT('Origin',(-15.,6.75,7.75));
#5290=CARTESIAN_POINT('',(-13.,2.775,7.75));
#5291=CARTESIAN_POINT('',(-15.,2.775,7.75));
#5292=CARTESIAN_POINT('',(-13.,-2.775,7.75));
#5293=CARTESIAN_POINT('',(-13.,2.775,7.75));
#5294=CARTESIAN_POINT('',(-15.,-2.775,7.75));
#5295=CARTESIAN_POINT('',(14.,-6.75,7.75));
#5296=CARTESIAN_POINT('',(-15.,-6.75,7.75));
#5297=CARTESIAN_POINT('',(14.,6.75,7.75));
#5298=CARTESIAN_POINT('',(14.,6.75,7.75));
#5299=CARTESIAN_POINT('',(-15.,6.75,7.75));
#5300=CARTESIAN_POINT('Origin',(15.,6.75,-7.75));
#5301=CARTESIAN_POINT('',(15.,6.75,6.75));
#5302=CARTESIAN_POINT('',(15.,6.75,-6.75));
#5303=CARTESIAN_POINT('',(15.,6.75,-7.75));
#5304=CARTESIAN_POINT('',(15.,-6.75,6.75));
#5305=CARTESIAN_POINT('',(15.,6.75,6.75));
#5306=CARTESIAN_POINT('',(15.,-6.75,-6.75));
#5307=CARTESIAN_POINT('',(15.,-6.75,-7.75));
#5308=CARTESIAN_POINT('',(15.,6.75,-6.75));
#5309=CARTESIAN_POINT('Origin',(-15.,6.75,-7.75));
#5310=CARTESIAN_POINT('',(-13.,-2.775,-7.75));
#5311=CARTESIAN_POINT('',(-13.,2.775,-7.75));
#5312=CARTESIAN_POINT('',(-13.,2.775,-7.75));
#5313=CARTESIAN_POINT('',(-15.,2.775,-7.75));
#5314=CARTESIAN_POINT('',(14.,6.75,-7.75));
#5315=CARTESIAN_POINT('',(-15.,6.75,-7.75));
#5316=CARTESIAN_POINT('',(14.,-6.75,-7.75));
#5317=CARTESIAN_POINT('',(14.,6.75,-7.75));
#5318=CARTESIAN_POINT('',(-15.,-6.75,-7.75));
#5319=CARTESIAN_POINT('',(-15.,-2.775,-7.75));
#5320=CARTESIAN_POINT('Origin',(0.,6.75,0.));
#5321=CARTESIAN_POINT('Origin',(14.,6.75,6.75));
#5322=CARTESIAN_POINT('Origin',(14.,6.75,-6.75));
#5323=CARTESIAN_POINT('',(13.6,6.75,-6.55));
#5324=CARTESIAN_POINT('',(-15.,6.75,-6.55));
#5325=CARTESIAN_POINT('',(13.8,6.75,-6.35));
#5326=CARTESIAN_POINT('Origin',(13.6,6.75,-6.35));
#5327=CARTESIAN_POINT('',(13.8,6.75,6.34999999999999));
#5328=CARTESIAN_POINT('',(13.8,6.75,6.54999999999999));
#5329=CARTESIAN_POINT('',(13.6,6.75,6.54999999999999));
#5330=CARTESIAN_POINT('Origin',(13.6,6.75,6.34999999999999));
#5331=CARTESIAN_POINT('',(-15.,6.75,6.55));
#5332=CARTESIAN_POINT('Origin',(0.,-6.75,0.));
#5333=CARTESIAN_POINT('Origin',(14.,-6.75,6.75));
#5334=CARTESIAN_POINT('',(13.6,-6.75,6.54999999999999));
#5335=CARTESIAN_POINT('',(-15.,-6.75,6.55));
#5336=CARTESIAN_POINT('',(13.8,-6.75,6.34999999999999));
#5337=CARTESIAN_POINT('Origin',(13.6,-6.75,6.34999999999999));
#5338=CARTESIAN_POINT('',(13.8,-6.75,-6.35));
#5339=CARTESIAN_POINT('',(13.8,-6.75,6.54999999999999));
#5340=CARTESIAN_POINT('',(13.6,-6.75,-6.55));
#5341=CARTESIAN_POINT('Origin',(13.6,-6.75,-6.35));
#5342=CARTESIAN_POINT('',(-15.,-6.75,-6.55));
#5343=CARTESIAN_POINT('Origin',(14.,-6.75,-6.75));
#5344=CARTESIAN_POINT('Origin',(-15.,-6.75,-6.55));
#5345=CARTESIAN_POINT('',(-13.,2.775,-6.55));
#5346=CARTESIAN_POINT('',(-15.,2.775,-6.55));
#5347=CARTESIAN_POINT('',(-13.,-2.775,-6.55));
#5348=CARTESIAN_POINT('',(-13.,-6.75,-6.55));
#5349=CARTESIAN_POINT('',(-15.,-2.775,-6.55));
#5350=CARTESIAN_POINT('',(13.6,6.75,-6.55));
#5351=CARTESIAN_POINT('Origin',(13.8,-6.75,6.54999999999999));
#5352=CARTESIAN_POINT('',(13.8,6.75,6.34999999999999));
#5353=CARTESIAN_POINT('',(13.8,-6.75,-6.35));
#5354=CARTESIAN_POINT('Origin',(-15.,-6.75,6.55));
#5355=CARTESIAN_POINT('',(-13.,-2.775,6.55));
#5356=CARTESIAN_POINT('',(-13.,2.775,6.55));
#5357=CARTESIAN_POINT('',(-13.,-6.75,6.55));
#5358=CARTESIAN_POINT('',(-15.,2.775,6.55));
#5359=CARTESIAN_POINT('',(13.6,-6.75,6.54999999999999));
#5360=CARTESIAN_POINT('',(-15.,-2.775,6.55));
#5361=CARTESIAN_POINT('Origin',(14.,6.75,6.75));
#5362=CARTESIAN_POINT('Origin',(14.,6.75,-6.75));
#5363=CARTESIAN_POINT('Origin',(13.6,-6.75,6.34999999999999));
#5364=CARTESIAN_POINT('Origin',(13.6,-6.75,-6.35));
#5365=CARTESIAN_POINT('Origin',(-15.,-2.775,-7.75));
#5366=CARTESIAN_POINT('',(-13.,-2.775,-7.75));
#5367=CARTESIAN_POINT('Origin',(-13.,2.775,-7.75));
#5368=CARTESIAN_POINT('',(-13.,2.775,-7.75));
#5369=CARTESIAN_POINT('Origin',(-15.,2.775,-7.75));
#5370=CARTESIAN_POINT('Origin',(-15.,2.775,-7.75));
#5371=CARTESIAN_POINT('',(-13.,2.775,-7.75));
#5372=CARTESIAN_POINT('Origin',(-13.,2.775,-7.75));
#5373=CARTESIAN_POINT('',(-13.,-2.775,-7.75));
#5374=CARTESIAN_POINT('Origin',(-15.,-2.775,-7.75));
#10531=UNCERTAINTY_MEASURE_WITH_UNIT(LENGTH_MEASURE(0.01),#10552,
'DISTANCE_ACCURACY_VALUE',
'Maximum model space distance between geometric entities at asserted c
onnectivities');
#10540=UNCERTAINTY_MEASURE_WITH_UNIT(LENGTH_MEASURE(0.01),#10552,
'DISTANCE_ACCURACY_VALUE',
'Maximum model space distance between geometric entities at asserted c
onnectivities');
#10542=(
GEOMETRIC_REPRESENTATION_CONTEXT(3)
GLOBAL_UNCERTAINTY_ASSIGNED_CONTEXT((#10531))
GLOBAL_UNIT_ASSIGNED_CONTEXT((#10552,#10554,#10555))
REPRESENTATION_CONTEXT('','3D')
);
#10551=(
GEOMETRIC_REPRESENTATION_CONTEXT(3)
GLOBAL_UNCERTAINTY_ASSIGNED_CONTEXT((#10540))
GLOBAL_UNIT_ASSIGNED_CONTEXT((#10552,#10554,#10555))
REPRESENTATION_CONTEXT('','3D')
);
#10552=(
LENGTH_UNIT()
NAMED_UNIT(*)
SI_UNIT(.MILLI.,.METRE.)
);
#10554=(
NAMED_UNIT(*)
PLANE_ANGLE_UNIT()
SI_UNIT($,.RADIAN.)
);
#10555=(
NAMED_UNIT(*)
SI_UNIT($,.STERADIAN.)
SOLID_ANGLE_UNIT()
);
#10557=SHAPE_DEFINITION_REPRESENTATION(#10567,#10586);
#10567=PRODUCT_DEFINITION_SHAPE('',$,#10597);
#10586=SHAPE_REPRESENTATION('',(#3537),#10542);
#10595=PRODUCT_DEFINITION_CONTEXT('part definition',#10627,'design');
#10597=PRODUCT_DEFINITION('Housing','Housing',#10607,#10595);
#10607=PRODUCT_DEFINITION_FORMATION('',$,#10630);
#10627=APPLICATION_CONTEXT(
'Core Data for Automotive Mechanical Design Process');
#10628=PRODUCT_CONTEXT('part definition',#10627,'mechanical');
#10630=PRODUCT('Housing','Housing','Housing',(#10628));
#10640=PRESENTATION_STYLE_ASSIGNMENT((#10647));
#10647=SURFACE_STYLE_USAGE(.BOTH.,#10654);
#10654=SURFACE_SIDE_STYLE('',(#10661));
#10661=SURFACE_STYLE_FILL_AREA(#10668);
#10668=FILL_AREA_STYLE('Opaque(20,51,87)',(#10675));
#10675=FILL_AREA_STYLE_COLOUR('Opaque(20,51,87)',#10682);
#10682=COLOUR_RGB('Opaque(20,51,87)',0.0784313725490196,0.2,0.341176470588235);
ENDSEC;
END-ISO-10303-21;
